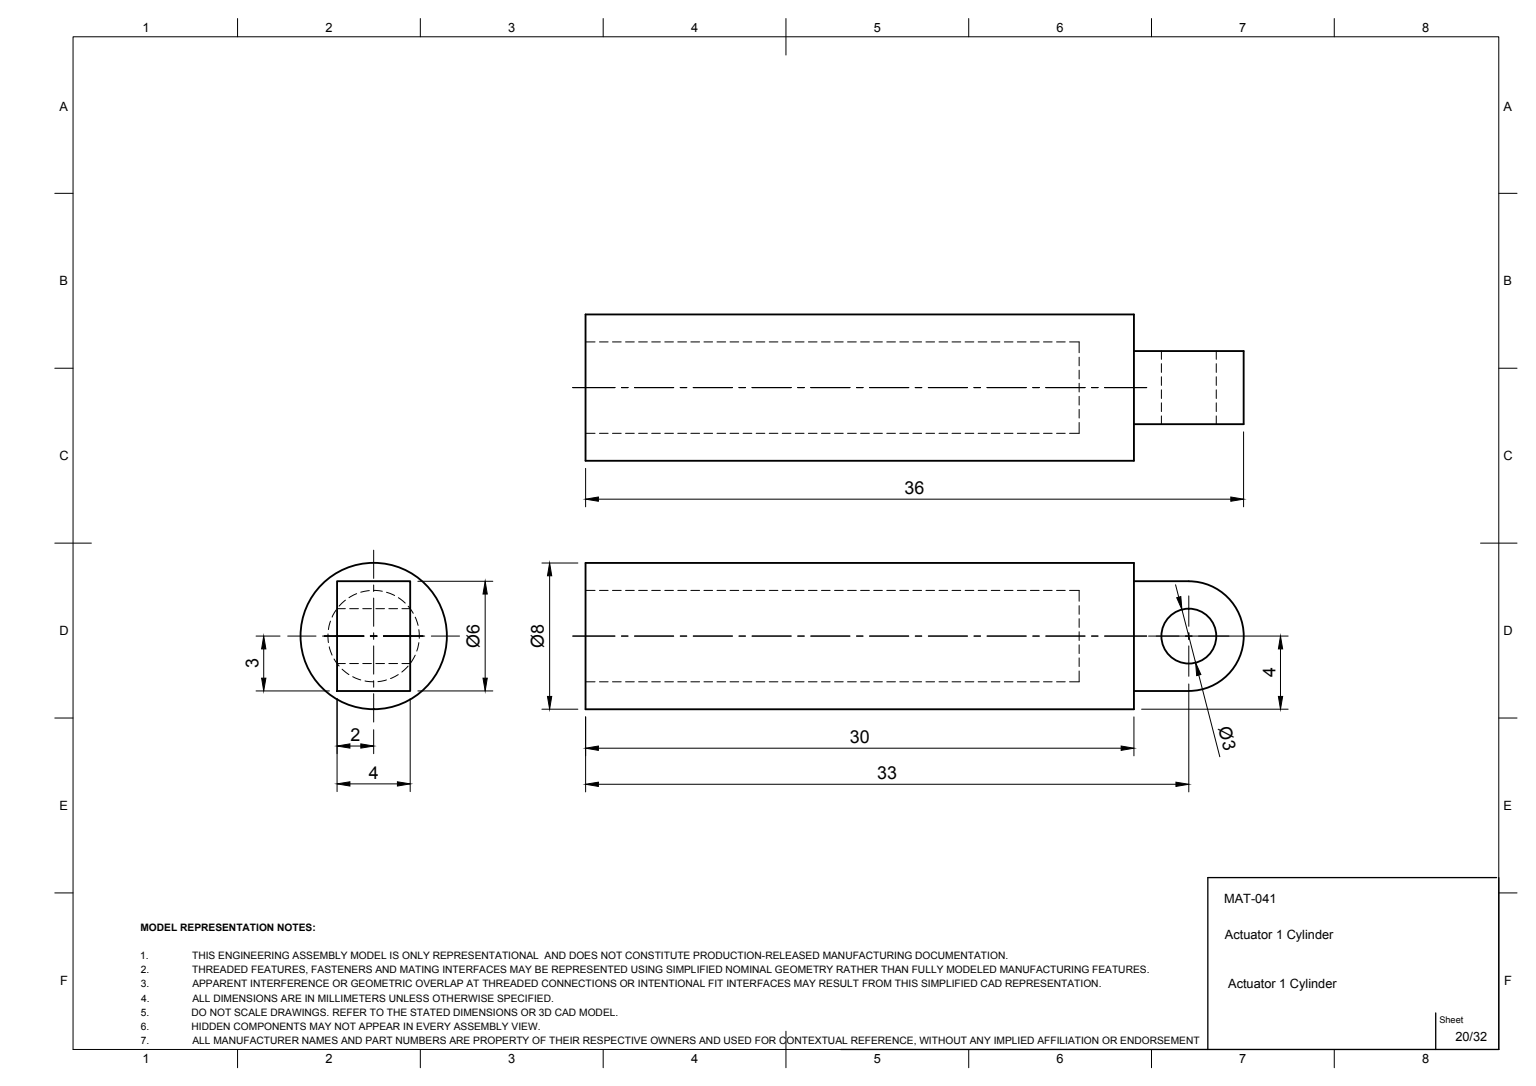
ISO-10303-21;
HEADER;
/* Generated by software containing ST-Developer
 * from STEP Tools, Inc. (www.steptools.com) 
 */

FILE_DESCRIPTION(
/* description */ ('STEP AP214'),
/* implementation_level */ '2;1');

FILE_NAME(
/* name */ 'Actuator 1 Cylinder.step',
/* time_stamp */ '2026-11-14T21:57:47-08:00',
/* author */ (''),
/* organization */ (''),
/* preprocessor_version */ 'ST-DEVELOPER v20.2',
/* originating_system */ 'Autodesk Translation Framework v15.17.0.0',
/* authorisation */ '');

FILE_SCHEMA (('AUTOMOTIVE_DESIGN { 1 0 10303 214 3 1 1 }'));
ENDSEC;

DATA;
#10=MECHANICAL_DESIGN_GEOMETRIC_PRESENTATION_REPRESENTATION('',(#256),#13199);
#220=SHAPE_REPRESENTATION_RELATIONSHIP('SRR','None',#13291,#238);
#238=ADVANCED_BREP_SHAPE_REPRESENTATION('',(#274),#13187);
#256=STYLED_ITEM('',(#13410),#274);
#274=MANIFOLD_SOLID_BREP('Body1',#6851);
#338=FACE_BOUND('',#2487,.T.);
#339=FACE_BOUND('',#2489,.T.);
#340=FACE_BOUND('',#2491,.T.);
#341=FACE_BOUND('',#2494,.T.);
#511=PLANE('',#7542);
#512=PLANE('',#7543);
#513=PLANE('',#7544);
#514=PLANE('',#7546);
#515=PLANE('',#7547);
#516=PLANE('',#7549);
#517=PLANE('',#7551);
#910=LINE('',#11772,#1428);
#911=LINE('',#11778,#1429);
#912=LINE('',#11784,#1430);
#913=LINE('',#11789,#1431);
#914=LINE('',#11791,#1432);
#915=LINE('',#11793,#1433);
#916=LINE('',#11794,#1434);
#917=LINE('',#11800,#1435);
#918=LINE('',#11801,#1436);
#919=LINE('',#11804,#1437);
#920=LINE('',#11805,#1438);
#921=LINE('',#11808,#1439);
#922=LINE('',#11811,#1440);
#1428=VECTOR('',#9079,2.5);
#1429=VECTOR('',#9086,1.5);
#1430=VECTOR('',#9093,4.);
#1431=VECTOR('',#9098,1000.);
#1432=VECTOR('',#9099,1000.);
#1433=VECTOR('',#9100,1000.);
#1434=VECTOR('',#9101,1000.);
#1435=VECTOR('',#9108,1000.);
#1436=VECTOR('',#9109,1000.);
#1437=VECTOR('',#9112,1000.);
#1438=VECTOR('',#9113,1000.);
#1439=VECTOR('',#9116,1000.);
#1440=VECTOR('',#9121,1000.);
#1744=CYLINDRICAL_SURFACE('',#7533,2.5);
#1745=CYLINDRICAL_SURFACE('',#7536,1.5);
#1746=CYLINDRICAL_SURFACE('',#7539,4.);
#1747=CYLINDRICAL_SURFACE('',#7550,3.);
#2038=FACE_OUTER_BOUND('',#2483,.T.);
#2039=FACE_OUTER_BOUND('',#2484,.T.);
#2040=FACE_OUTER_BOUND('',#2485,.T.);
#2041=FACE_OUTER_BOUND('',#2486,.T.);
#2042=FACE_OUTER_BOUND('',#2488,.T.);
#2043=FACE_OUTER_BOUND('',#2490,.T.);
#2044=FACE_OUTER_BOUND('',#2492,.T.);
#2045=FACE_OUTER_BOUND('',#2493,.T.);
#2046=FACE_OUTER_BOUND('',#2495,.T.);
#2047=FACE_OUTER_BOUND('',#2496,.T.);
#2048=FACE_OUTER_BOUND('',#2497,.T.);
#2483=EDGE_LOOP('',(#5706,#5707,#5708,#5709));
#2484=EDGE_LOOP('',(#5710,#5711,#5712,#5713));
#2485=EDGE_LOOP('',(#5714,#5715,#5716,#5717));
#2486=EDGE_LOOP('',(#5718));
#2487=EDGE_LOOP('',(#5719,#5720,#5721,#5722));
#2488=EDGE_LOOP('',(#5723));
#2489=EDGE_LOOP('',(#5724));
#2490=EDGE_LOOP('',(#5725,#5726,#5727,#5728));
#2491=EDGE_LOOP('',(#5729));
#2492=EDGE_LOOP('',(#5730,#5731,#5732,#5733));
#2493=EDGE_LOOP('',(#5734,#5735,#5736,#5737));
#2494=EDGE_LOOP('',(#5738));
#2495=EDGE_LOOP('',(#5739,#5740,#5741,#5742));
#2496=EDGE_LOOP('',(#5743,#5744,#5745,#5746));
#2497=EDGE_LOOP('',(#5747));
#2889=CIRCLE('',#7534,2.5);
#2890=CIRCLE('',#7535,2.5);
#2891=CIRCLE('',#7537,1.5);
#2892=CIRCLE('',#7538,1.5);
#2893=CIRCLE('',#7540,4.);
#2894=CIRCLE('',#7541,4.);
#2895=CIRCLE('',#7545,3.);
#2896=CIRCLE('',#7548,3.);
#3370=VERTEX_POINT('',#11769);
#3371=VERTEX_POINT('',#11771);
#3372=VERTEX_POINT('',#11775);
#3373=VERTEX_POINT('',#11777);
#3374=VERTEX_POINT('',#11781);
#3375=VERTEX_POINT('',#11783);
#3376=VERTEX_POINT('',#11787);
#3377=VERTEX_POINT('',#11788);
#3378=VERTEX_POINT('',#11790);
#3379=VERTEX_POINT('',#11792);
#3380=VERTEX_POINT('',#11797);
#3381=VERTEX_POINT('',#11798);
#3382=VERTEX_POINT('',#11803);
#3383=VERTEX_POINT('',#11807);
#4190=EDGE_CURVE('',#3370,#3370,#2889,.T.);
#4191=EDGE_CURVE('',#3370,#3371,#910,.T.);
#4192=EDGE_CURVE('',#3371,#3371,#2890,.T.);
#4193=EDGE_CURVE('',#3372,#3372,#2891,.T.);
#4194=EDGE_CURVE('',#3372,#3373,#911,.T.);
#4195=EDGE_CURVE('',#3373,#3373,#2892,.T.);
#4196=EDGE_CURVE('',#3374,#3374,#2893,.T.);
#4197=EDGE_CURVE('',#3374,#3375,#912,.T.);
#4198=EDGE_CURVE('',#3375,#3375,#2894,.T.);
#4199=EDGE_CURVE('',#3376,#3377,#913,.T.);
#4200=EDGE_CURVE('',#3378,#3376,#914,.T.);
#4201=EDGE_CURVE('',#3379,#3378,#915,.T.);
#4202=EDGE_CURVE('',#3377,#3379,#916,.T.);
#4203=EDGE_CURVE('',#3380,#3381,#2895,.T.);
#4204=EDGE_CURVE('',#3381,#3376,#917,.T.);
#4205=EDGE_CURVE('',#3380,#3377,#918,.T.);
#4206=EDGE_CURVE('',#3382,#3379,#919,.T.);
#4207=EDGE_CURVE('',#3382,#3380,#920,.T.);
#4208=EDGE_CURVE('',#3383,#3378,#921,.T.);
#4209=EDGE_CURVE('',#3383,#3382,#2896,.T.);
#4210=EDGE_CURVE('',#3381,#3383,#922,.T.);
#5706=ORIENTED_EDGE('',*,*,#4190,.F.);
#5707=ORIENTED_EDGE('',*,*,#4191,.T.);
#5708=ORIENTED_EDGE('',*,*,#4192,.T.);
#5709=ORIENTED_EDGE('',*,*,#4191,.F.);
#5710=ORIENTED_EDGE('',*,*,#4193,.F.);
#5711=ORIENTED_EDGE('',*,*,#4194,.T.);
#5712=ORIENTED_EDGE('',*,*,#4195,.T.);
#5713=ORIENTED_EDGE('',*,*,#4194,.F.);
#5714=ORIENTED_EDGE('',*,*,#4196,.T.);
#5715=ORIENTED_EDGE('',*,*,#4197,.T.);
#5716=ORIENTED_EDGE('',*,*,#4198,.F.);
#5717=ORIENTED_EDGE('',*,*,#4197,.F.);
#5718=ORIENTED_EDGE('',*,*,#4196,.F.);
#5719=ORIENTED_EDGE('',*,*,#4199,.F.);
#5720=ORIENTED_EDGE('',*,*,#4200,.F.);
#5721=ORIENTED_EDGE('',*,*,#4201,.F.);
#5722=ORIENTED_EDGE('',*,*,#4202,.F.);
#5723=ORIENTED_EDGE('',*,*,#4198,.T.);
#5724=ORIENTED_EDGE('',*,*,#4192,.F.);
#5725=ORIENTED_EDGE('',*,*,#4203,.T.);
#5726=ORIENTED_EDGE('',*,*,#4204,.T.);
#5727=ORIENTED_EDGE('',*,*,#4199,.T.);
#5728=ORIENTED_EDGE('',*,*,#4205,.F.);
#5729=ORIENTED_EDGE('',*,*,#4193,.T.);
#5730=ORIENTED_EDGE('',*,*,#4206,.F.);
#5731=ORIENTED_EDGE('',*,*,#4207,.T.);
#5732=ORIENTED_EDGE('',*,*,#4205,.T.);
#5733=ORIENTED_EDGE('',*,*,#4202,.T.);
#5734=ORIENTED_EDGE('',*,*,#4208,.F.);
#5735=ORIENTED_EDGE('',*,*,#4209,.T.);
#5736=ORIENTED_EDGE('',*,*,#4206,.T.);
#5737=ORIENTED_EDGE('',*,*,#4201,.T.);
#5738=ORIENTED_EDGE('',*,*,#4195,.F.);
#5739=ORIENTED_EDGE('',*,*,#4204,.F.);
#5740=ORIENTED_EDGE('',*,*,#4210,.T.);
#5741=ORIENTED_EDGE('',*,*,#4208,.T.);
#5742=ORIENTED_EDGE('',*,*,#4200,.T.);
#5743=ORIENTED_EDGE('',*,*,#4207,.F.);
#5744=ORIENTED_EDGE('',*,*,#4209,.F.);
#5745=ORIENTED_EDGE('',*,*,#4210,.F.);
#5746=ORIENTED_EDGE('',*,*,#4203,.F.);
#5747=ORIENTED_EDGE('',*,*,#4190,.T.);
#6690=ADVANCED_FACE('',(#2038),#1744,.F.);
#6691=ADVANCED_FACE('',(#2039),#1745,.F.);
#6692=ADVANCED_FACE('',(#2040),#1746,.T.);
#6693=ADVANCED_FACE('',(#2041,#338),#511,.F.);
#6694=ADVANCED_FACE('',(#2042,#339),#512,.T.);
#6695=ADVANCED_FACE('',(#2043,#340),#513,.F.);
#6696=ADVANCED_FACE('',(#2044),#514,.F.);
#6697=ADVANCED_FACE('',(#2045,#341),#515,.F.);
#6698=ADVANCED_FACE('',(#2046),#516,.F.);
#6699=ADVANCED_FACE('',(#2047),#1747,.T.);
#6700=ADVANCED_FACE('',(#2048),#517,.T.);
#6851=CLOSED_SHELL('',(#6690,#6691,#6692,#6693,#6694,#6695,#6696,#6697,
#6698,#6699,#6700));
#7532=AXIS2_PLACEMENT_3D('',#11767,#9073,#9074);
#7533=AXIS2_PLACEMENT_3D('',#11768,#9075,#9076);
#7534=AXIS2_PLACEMENT_3D('',#11770,#9077,#9078);
#7535=AXIS2_PLACEMENT_3D('',#11773,#9080,#9081);
#7536=AXIS2_PLACEMENT_3D('',#11774,#9082,#9083);
#7537=AXIS2_PLACEMENT_3D('',#11776,#9084,#9085);
#7538=AXIS2_PLACEMENT_3D('',#11779,#9087,#9088);
#7539=AXIS2_PLACEMENT_3D('',#11780,#9089,#9090);
#7540=AXIS2_PLACEMENT_3D('',#11782,#9091,#9092);
#7541=AXIS2_PLACEMENT_3D('',#11785,#9094,#9095);
#7542=AXIS2_PLACEMENT_3D('',#11786,#9096,#9097);
#7543=AXIS2_PLACEMENT_3D('',#11795,#9102,#9103);
#7544=AXIS2_PLACEMENT_3D('',#11796,#9104,#9105);
#7545=AXIS2_PLACEMENT_3D('',#11799,#9106,#9107);
#7546=AXIS2_PLACEMENT_3D('',#11802,#9110,#9111);
#7547=AXIS2_PLACEMENT_3D('',#11806,#9114,#9115);
#7548=AXIS2_PLACEMENT_3D('',#11809,#9117,#9118);
#7549=AXIS2_PLACEMENT_3D('',#11810,#9119,#9120);
#7550=AXIS2_PLACEMENT_3D('',#11812,#9122,#9123);
#7551=AXIS2_PLACEMENT_3D('',#11813,#9124,#9125);
#9073=DIRECTION('axis',(0.,0.,1.));
#9074=DIRECTION('refdir',(1.,0.,0.));
#9075=DIRECTION('center_axis',(0.,0.,1.));
#9076=DIRECTION('ref_axis',(1.,0.,0.));
#9077=DIRECTION('center_axis',(0.,0.,1.));
#9078=DIRECTION('ref_axis',(1.,0.,0.));
#9079=DIRECTION('',(0.,0.,1.));
#9080=DIRECTION('center_axis',(0.,0.,1.));
#9081=DIRECTION('ref_axis',(1.,0.,0.));
#9082=DIRECTION('center_axis',(1.,-1.0842021724855E-16,0.));
#9083=DIRECTION('ref_axis',(1.0842021724855E-16,1.,0.));
#9084=DIRECTION('center_axis',(1.,-7.2280144832367E-17,0.));
#9085=DIRECTION('ref_axis',(7.2280144832367E-17,1.,0.));
#9086=DIRECTION('',(1.,-1.0842021724855E-16,0.));
#9087=DIRECTION('center_axis',(1.,-1.0842021724855E-16,0.));
#9088=DIRECTION('ref_axis',(1.0842021724855E-16,1.,0.));
#9089=DIRECTION('center_axis',(0.,0.,-1.));
#9090=DIRECTION('ref_axis',(-1.,0.,0.));
#9091=DIRECTION('center_axis',(0.,0.,1.));
#9092=DIRECTION('ref_axis',(1.,0.,0.));
#9093=DIRECTION('',(0.,0.,1.));
#9094=DIRECTION('center_axis',(0.,0.,1.));
#9095=DIRECTION('ref_axis',(1.,0.,0.));
#9096=DIRECTION('center_axis',(0.,0.,1.));
#9097=DIRECTION('ref_axis',(1.,0.,0.));
#9098=DIRECTION('',(7.2280144832367E-17,1.,0.));
#9099=DIRECTION('',(-1.,0.,0.));
#9100=DIRECTION('',(-1.44560289664734E-16,-1.,0.));
#9101=DIRECTION('',(1.,0.,0.));
#9102=DIRECTION('center_axis',(0.,0.,1.));
#9103=DIRECTION('ref_axis',(1.,0.,0.));
#9104=DIRECTION('center_axis',(1.,-7.2280144832367E-17,0.));
#9105=DIRECTION('ref_axis',(7.2280144832367E-17,1.,0.));
#9106=DIRECTION('center_axis',(-1.,7.2280144832367E-17,0.));
#9107=DIRECTION('ref_axis',(7.22801448323669E-17,1.,0.));
#9108=DIRECTION('',(0.,0.,1.));
#9109=DIRECTION('',(0.,0.,1.));
#9110=DIRECTION('center_axis',(0.,-1.,0.));
#9111=DIRECTION('ref_axis',(0.,0.,-1.));
#9112=DIRECTION('',(0.,0.,1.));
#9113=DIRECTION('',(-1.,0.,0.));
#9114=DIRECTION('center_axis',(-1.,1.44560289664734E-16,0.));
#9115=DIRECTION('ref_axis',(-1.44560289664734E-16,-1.,0.));
#9116=DIRECTION('',(0.,0.,1.));
#9117=DIRECTION('center_axis',(1.,-1.44560289664734E-16,0.));
#9118=DIRECTION('ref_axis',(-1.44560289664734E-16,-1.,0.));
#9119=DIRECTION('center_axis',(0.,1.,0.));
#9120=DIRECTION('ref_axis',(0.,0.,1.));
#9121=DIRECTION('',(1.,0.,0.));
#9122=DIRECTION('center_axis',(-1.,0.,0.));
#9123=DIRECTION('ref_axis',(0.,1.22464679914735E-16,-1.));
#9124=DIRECTION('center_axis',(0.,0.,1.));
#9125=DIRECTION('ref_axis',(1.,0.,0.));
#11767=CARTESIAN_POINT('',(0.,0.,0.));
#11768=CARTESIAN_POINT('Origin',(0.,0.,3.));
#11769=CARTESIAN_POINT('',(-2.5,-3.06161699786838E-16,3.));
#11770=CARTESIAN_POINT('Origin',(0.,0.,3.));
#11771=CARTESIAN_POINT('',(-2.5,-3.06161699786838E-16,30.));
#11772=CARTESIAN_POINT('',(-2.5,-3.06161699786838E-16,3.));
#11773=CARTESIAN_POINT('Origin',(0.,0.,30.));
#11774=CARTESIAN_POINT('Origin',(-4.,4.33680868994202E-16,-3.));
#11775=CARTESIAN_POINT('',(-2.,-1.5,-3.));
#11776=CARTESIAN_POINT('Origin',(-2.,2.16840434497101E-16,-3.));
#11777=CARTESIAN_POINT('',(2.,-1.5,-3.));
#11778=CARTESIAN_POINT('',(-4.,-1.5,-3.));
#11779=CARTESIAN_POINT('Origin',(2.,-2.16840434497101E-16,-3.));
#11780=CARTESIAN_POINT('Origin',(0.,0.,30.));
#11781=CARTESIAN_POINT('',(4.,-4.89858719658941E-16,0.));
#11782=CARTESIAN_POINT('Origin',(0.,0.,0.));
#11783=CARTESIAN_POINT('',(4.,-4.89858719658941E-16,30.));
#11784=CARTESIAN_POINT('',(4.,-4.89858719658941E-16,30.));
#11785=CARTESIAN_POINT('Origin',(0.,0.,30.));
#11786=CARTESIAN_POINT('Origin',(0.,0.,0.));
#11787=CARTESIAN_POINT('',(-2.,-3.,0.));
#11788=CARTESIAN_POINT('',(-2.,3.,0.));
#11789=CARTESIAN_POINT('',(-2.,3.,0.));
#11790=CARTESIAN_POINT('',(2.,-3.,0.));
#11791=CARTESIAN_POINT('',(2.,-3.,0.));
#11792=CARTESIAN_POINT('',(2.,3.,0.));
#11793=CARTESIAN_POINT('',(2.,3.,0.));
#11794=CARTESIAN_POINT('',(2.,3.,0.));
#11795=CARTESIAN_POINT('Origin',(0.,0.,30.));
#11796=CARTESIAN_POINT('Origin',(-2.,3.,-6.));
#11797=CARTESIAN_POINT('',(-2.,3.,-3.));
#11798=CARTESIAN_POINT('',(-2.,-3.,-3.));
#11799=CARTESIAN_POINT('Origin',(-2.,0.,-3.));
#11800=CARTESIAN_POINT('',(-2.,-3.,-6.));
#11801=CARTESIAN_POINT('',(-2.,3.,-6.));
#11802=CARTESIAN_POINT('Origin',(2.,3.,-6.));
#11803=CARTESIAN_POINT('',(2.,3.,-3.));
#11804=CARTESIAN_POINT('',(2.,3.,-6.));
#11805=CARTESIAN_POINT('',(-2.,3.,-3.));
#11806=CARTESIAN_POINT('Origin',(2.,3.,-6.));
#11807=CARTESIAN_POINT('',(2.,-3.,-3.));
#11808=CARTESIAN_POINT('',(2.,-3.,-6.));
#11809=CARTESIAN_POINT('Origin',(2.,0.,-3.));
#11810=CARTESIAN_POINT('Origin',(2.,-3.,-6.));
#11811=CARTESIAN_POINT('',(2.,-3.,-3.));
#11812=CARTESIAN_POINT('Origin',(0.,0.,-3.));
#11813=CARTESIAN_POINT('Origin',(0.,0.,3.));
#13161=UNCERTAINTY_MEASURE_WITH_UNIT(LENGTH_MEASURE(0.01),#13200,
'DISTANCE_ACCURACY_VALUE',
'Maximum model space distance between geometric entities at asserted c
onnectivities');
#13173=UNCERTAINTY_MEASURE_WITH_UNIT(LENGTH_MEASURE(0.01),#13200,
'DISTANCE_ACCURACY_VALUE',
'Maximum model space distance between geometric entities at asserted c
onnectivities');
#13187=(
GEOMETRIC_REPRESENTATION_CONTEXT(3)
GLOBAL_UNCERTAINTY_ASSIGNED_CONTEXT((#13161))
GLOBAL_UNIT_ASSIGNED_CONTEXT((#13200,#13202,#13203))
REPRESENTATION_CONTEXT('','3D')
);
#13199=(
GEOMETRIC_REPRESENTATION_CONTEXT(3)
GLOBAL_UNCERTAINTY_ASSIGNED_CONTEXT((#13173))
GLOBAL_UNIT_ASSIGNED_CONTEXT((#13200,#13202,#13203))
REPRESENTATION_CONTEXT('','3D')
);
#13200=(
LENGTH_UNIT()
NAMED_UNIT(*)
SI_UNIT(.MILLI.,.METRE.)
);
#13202=(
NAMED_UNIT(*)
PLANE_ANGLE_UNIT()
SI_UNIT($,.RADIAN.)
);
#13203=(
NAMED_UNIT(*)
SI_UNIT($,.STERADIAN.)
SOLID_ANGLE_UNIT()
);
#13217=SHAPE_DEFINITION_REPRESENTATION(#13246,#13291);
#13246=PRODUCT_DEFINITION_SHAPE('',$,#13317);
#13291=SHAPE_REPRESENTATION('',(#7532),#13187);
#13303=PRODUCT_DEFINITION_CONTEXT('part definition',#13380,'design');
#13317=PRODUCT_DEFINITION('Actuator 1 Cylinder','Actuator 1 Cylinder',#13342,
#13303);
#13342=PRODUCT_DEFINITION_FORMATION('',$,#13395);
#13380=APPLICATION_CONTEXT(
'Core Data for Automotive Mechanical Design Process');
#13381=PRODUCT_CONTEXT('part definition',#13380,'mechanical');
#13395=PRODUCT('Actuator 1 Cylinder','Actuator 1 Cylinder',$,(#13381));
#13410=PRESENTATION_STYLE_ASSIGNMENT((#13415));
#13415=SURFACE_STYLE_USAGE(.BOTH.,#13420);
#13420=SURFACE_SIDE_STYLE('',(#13425));
#13425=SURFACE_STYLE_FILL_AREA(#13430);
#13430=FILL_AREA_STYLE('Opaque(227,224,212)',(#13435));
#13435=FILL_AREA_STYLE_COLOUR('Opaque(227,224,212)',#13440);
#13440=COLOUR_RGB('Opaque(227,224,212)',0.890196078431372,0.87843137254902,
0.831372549019608);
ENDSEC;
END-ISO-10303-21;
